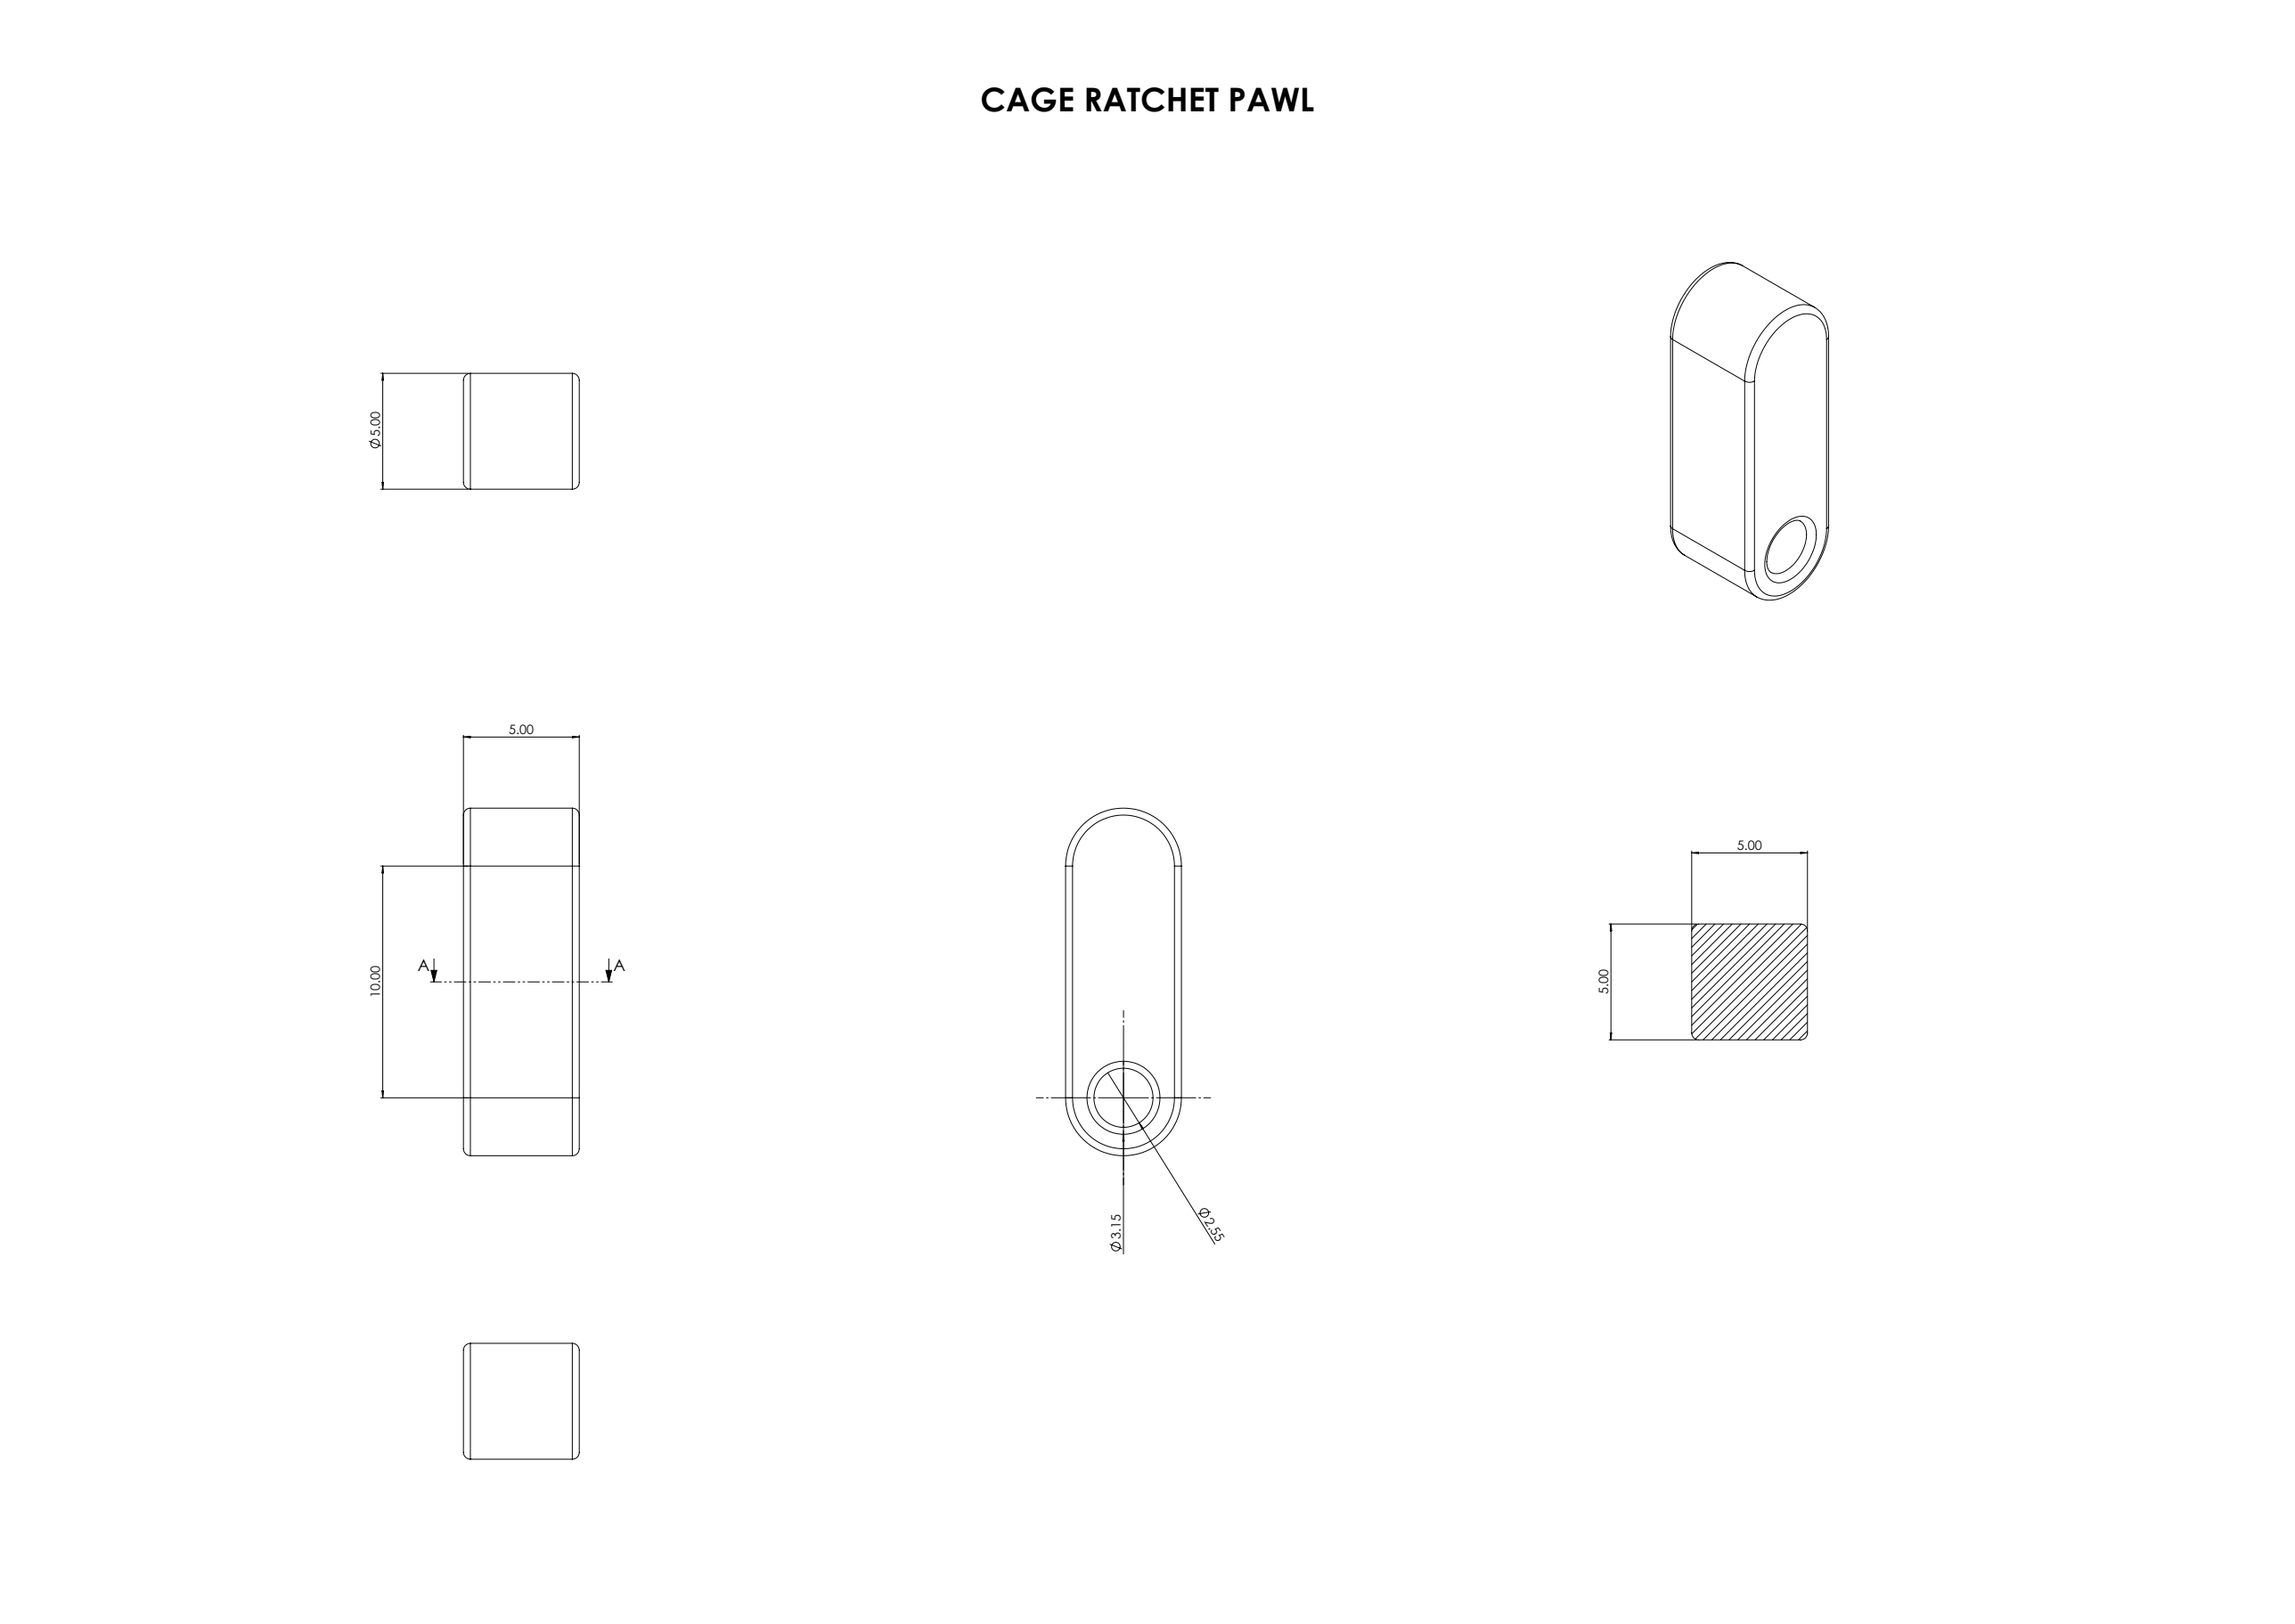
ISO-10303-21;
HEADER;
/* Generated by software containing ST-Developer
 * from STEP Tools, Inc. (www.steptools.com) 
 */

FILE_DESCRIPTION(
/* description */ (''),
/* implementation_level */ '2;1');

FILE_NAME(
/* name */ '05_Cage_Ratchet_Pawl.step',
/* time_stamp */ '2026-10-11T13:00:10-07:00',
/* author */ (''),
/* organization */ (''),
/* preprocessor_version */ 'ST-DEVELOPER v20.2',
/* originating_system */ 'Autodesk Translation Framework v15.15.0.0',
/* authorisation */ '');

FILE_SCHEMA (('AUTOMOTIVE_DESIGN { 1 0 10303 214 3 1 1 }'));
ENDSEC;

DATA;
#10=MECHANICAL_DESIGN_GEOMETRIC_PRESENTATION_REPRESENTATION('',(#362),#65563);
#149=TOROIDAL_SURFACE('',#21705,2.2,0.3);
#150=TOROIDAL_SURFACE('',#21711,2.2,0.3);
#151=TOROIDAL_SURFACE('',#21722,2.2,0.3);
#152=TOROIDAL_SURFACE('',#21728,2.2,0.3);
#153=TOROIDAL_SURFACE('',#21733,1.575,0.3);
#154=TOROIDAL_SURFACE('',#21739,1.575,0.3);
#340=SHAPE_REPRESENTATION_RELATIONSHIP('SRR','None',#65618,#351);
#351=ADVANCED_BREP_SHAPE_REPRESENTATION('',(#373),#65556);
#362=STYLED_ITEM('',(#65781),#373);
#373=MANIFOLD_SOLID_BREP('Body1',#20012);
#976=PLANE('',#21716);
#977=PLANE('',#21717);
#978=PLANE('',#21731);
#979=PLANE('',#21741);
#1118=FACE_BOUND('',#3216,.T.);
#1119=FACE_BOUND('',#3223,.T.);
#1987=FACE_OUTER_BOUND('',#3209,.T.);
#1988=FACE_OUTER_BOUND('',#3210,.T.);
#1989=FACE_OUTER_BOUND('',#3211,.T.);
#1990=FACE_OUTER_BOUND('',#3212,.T.);
#1991=FACE_OUTER_BOUND('',#3213,.T.);
#1992=FACE_OUTER_BOUND('',#3214,.T.);
#1993=FACE_OUTER_BOUND('',#3215,.T.);
#1994=FACE_OUTER_BOUND('',#3217,.T.);
#1995=FACE_OUTER_BOUND('',#3218,.T.);
#1996=FACE_OUTER_BOUND('',#3219,.T.);
#1997=FACE_OUTER_BOUND('',#3220,.T.);
#1998=FACE_OUTER_BOUND('',#3221,.T.);
#1999=FACE_OUTER_BOUND('',#3222,.T.);
#2000=FACE_OUTER_BOUND('',#3224,.T.);
#2001=FACE_OUTER_BOUND('',#3225,.T.);
#2002=FACE_OUTER_BOUND('',#3226,.T.);
#2003=FACE_OUTER_BOUND('',#3227,.T.);
#3209=EDGE_LOOP('',(#16744,#16745,#16746,#16747));
#3210=EDGE_LOOP('',(#16748,#16749,#16750,#16751));
#3211=EDGE_LOOP('',(#16752,#16753,#16754,#16755));
#3212=EDGE_LOOP('',(#16756,#16757,#16758,#16759));
#3213=EDGE_LOOP('',(#16760,#16761,#16762,#16763));
#3214=EDGE_LOOP('',(#16764,#16765,#16766,#16767));
#3215=EDGE_LOOP('',(#16768,#16769,#16770,#16771));
#3216=EDGE_LOOP('',(#16772));
#3217=EDGE_LOOP('',(#16773,#16774,#16775,#16776));
#3218=EDGE_LOOP('',(#16777,#16778,#16779,#16780));
#3219=EDGE_LOOP('',(#16781,#16782,#16783,#16784));
#3220=EDGE_LOOP('',(#16785,#16786,#16787,#16788));
#3221=EDGE_LOOP('',(#16789,#16790,#16791,#16792));
#3222=EDGE_LOOP('',(#16793,#16794,#16795,#16796));
#3223=EDGE_LOOP('',(#16797));
#3224=EDGE_LOOP('',(#16798,#16799,#16800,#16801));
#3225=EDGE_LOOP('',(#16802,#16803,#16804,#16805,#16806));
#3226=EDGE_LOOP('',(#16807,#16808,#16809,#16810,#16811));
#3227=EDGE_LOOP('',(#16812,#16813,#16814,#16815));
#4320=CIRCLE('',#21703,0.3);
#4321=CIRCLE('',#21704,0.3);
#4322=CIRCLE('',#21706,0.3);
#4323=CIRCLE('',#21707,2.2);
#4324=CIRCLE('',#21708,2.5);
#4325=CIRCLE('',#21710,0.3);
#4326=CIRCLE('',#21712,2.2);
#4327=CIRCLE('',#21713,2.5);
#4328=CIRCLE('',#21715,2.5);
#4329=CIRCLE('',#21718,1.575);
#4330=CIRCLE('',#21720,0.3);
#4331=CIRCLE('',#21721,0.3);
#4332=CIRCLE('',#21723,0.3);
#4333=CIRCLE('',#21724,2.2);
#4334=CIRCLE('',#21725,2.5);
#4335=CIRCLE('',#21727,0.3);
#4336=CIRCLE('',#21729,2.2);
#4337=CIRCLE('',#21732,1.575);
#4338=CIRCLE('',#21734,0.3);
#4339=CIRCLE('',#21735,1.275);
#4340=CIRCLE('',#21737,1.275);
#4341=CIRCLE('',#21738,1.275);
#4342=CIRCLE('',#21740,0.3);
#6010=LINE('',#61877,#6902);
#6011=LINE('',#61880,#6903);
#6012=LINE('',#61891,#6904);
#6013=LINE('',#61892,#6905);
#6014=LINE('',#61898,#6906);
#6015=LINE('',#61901,#6907);
#6016=LINE('',#61904,#6908);
#6017=LINE('',#61905,#6909);
#6018=LINE('',#61914,#6910);
#6019=LINE('',#61924,#6911);
#6020=LINE('',#61925,#6912);
#6021=LINE('',#61929,#6913);
#6022=LINE('',#61939,#6914);
#6902=VECTOR('',#26097,10.);
#6903=VECTOR('',#26100,10.);
#6904=VECTOR('',#26113,10.);
#6905=VECTOR('',#26114,10.);
#6906=VECTOR('',#26123,10.);
#6907=VECTOR('',#26126,10.);
#6908=VECTOR('',#26129,10.);
#6909=VECTOR('',#26130,10.);
#6910=VECTOR('',#26141,10.);
#6911=VECTOR('',#26154,10.);
#6912=VECTOR('',#26155,10.);
#6913=VECTOR('',#26162,10.);
#6914=VECTOR('',#26175,1.275);
#8661=VERTEX_POINT('',#61873);
#8662=VERTEX_POINT('',#61874);
#8663=VERTEX_POINT('',#61876);
#8664=VERTEX_POINT('',#61878);
#8665=VERTEX_POINT('',#61882);
#8666=VERTEX_POINT('',#61883);
#8667=VERTEX_POINT('',#61888);
#8668=VERTEX_POINT('',#61889);
#8669=VERTEX_POINT('',#61897);
#8670=VERTEX_POINT('',#61899);
#8671=VERTEX_POINT('',#61903);
#8672=VERTEX_POINT('',#61907);
#8673=VERTEX_POINT('',#61910);
#8674=VERTEX_POINT('',#61912);
#8675=VERTEX_POINT('',#61916);
#8676=VERTEX_POINT('',#61917);
#8677=VERTEX_POINT('',#61922);
#8678=VERTEX_POINT('',#61931);
#8679=VERTEX_POINT('',#61934);
#8680=VERTEX_POINT('',#61938);
#8681=VERTEX_POINT('',#61940);
#11405=EDGE_CURVE('',#8661,#8662,#4320,.T.);
#11406=EDGE_CURVE('',#8662,#8663,#6010,.T.);
#11407=EDGE_CURVE('',#8663,#8664,#4321,.T.);
#11408=EDGE_CURVE('',#8664,#8661,#6011,.T.);
#11409=EDGE_CURVE('',#8665,#8666,#4322,.T.);
#11410=EDGE_CURVE('',#8666,#8664,#4323,.T.);
#11411=EDGE_CURVE('',#8663,#8665,#4324,.T.);
#11412=EDGE_CURVE('',#8667,#8668,#4325,.T.);
#11413=EDGE_CURVE('',#8668,#8666,#6012,.T.);
#11414=EDGE_CURVE('',#8665,#8667,#6013,.T.);
#11415=EDGE_CURVE('',#8661,#8668,#4326,.T.);
#11416=EDGE_CURVE('',#8667,#8662,#4327,.T.);
#11417=EDGE_CURVE('',#8669,#8663,#6014,.T.);
#11418=EDGE_CURVE('',#8670,#8669,#4328,.T.);
#11419=EDGE_CURVE('',#8670,#8665,#6015,.T.);
#11420=EDGE_CURVE('',#8671,#8662,#6016,.T.);
#11421=EDGE_CURVE('',#8669,#8671,#6017,.T.);
#11422=EDGE_CURVE('',#8672,#8672,#4329,.T.);
#11423=EDGE_CURVE('',#8673,#8669,#4330,.T.);
#11424=EDGE_CURVE('',#8671,#8674,#4331,.T.);
#11425=EDGE_CURVE('',#8674,#8673,#6018,.T.);
#11426=EDGE_CURVE('',#8675,#8676,#4332,.T.);
#11427=EDGE_CURVE('',#8676,#8674,#4333,.T.);
#11428=EDGE_CURVE('',#8671,#8675,#4334,.T.);
#11429=EDGE_CURVE('',#8670,#8677,#4335,.T.);
#11430=EDGE_CURVE('',#8677,#8676,#6019,.T.);
#11431=EDGE_CURVE('',#8675,#8670,#6020,.T.);
#11432=EDGE_CURVE('',#8673,#8677,#4336,.T.);
#11433=EDGE_CURVE('',#8675,#8667,#6021,.T.);
#11434=EDGE_CURVE('',#8678,#8678,#4337,.T.);
#11435=EDGE_CURVE('',#8678,#8679,#4338,.T.);
#11436=EDGE_CURVE('',#8679,#8679,#4339,.T.);
#11437=EDGE_CURVE('',#8679,#8680,#6022,.T.);
#11438=EDGE_CURVE('',#8681,#8680,#4340,.T.);
#11439=EDGE_CURVE('',#8680,#8681,#4341,.T.);
#11440=EDGE_CURVE('',#8672,#8681,#4342,.T.);
#16744=ORIENTED_EDGE('',*,*,#11405,.T.);
#16745=ORIENTED_EDGE('',*,*,#11406,.T.);
#16746=ORIENTED_EDGE('',*,*,#11407,.T.);
#16747=ORIENTED_EDGE('',*,*,#11408,.T.);
#16748=ORIENTED_EDGE('',*,*,#11409,.T.);
#16749=ORIENTED_EDGE('',*,*,#11410,.T.);
#16750=ORIENTED_EDGE('',*,*,#11407,.F.);
#16751=ORIENTED_EDGE('',*,*,#11411,.T.);
#16752=ORIENTED_EDGE('',*,*,#11412,.T.);
#16753=ORIENTED_EDGE('',*,*,#11413,.T.);
#16754=ORIENTED_EDGE('',*,*,#11409,.F.);
#16755=ORIENTED_EDGE('',*,*,#11414,.T.);
#16756=ORIENTED_EDGE('',*,*,#11405,.F.);
#16757=ORIENTED_EDGE('',*,*,#11415,.T.);
#16758=ORIENTED_EDGE('',*,*,#11412,.F.);
#16759=ORIENTED_EDGE('',*,*,#11416,.T.);
#16760=ORIENTED_EDGE('',*,*,#11411,.F.);
#16761=ORIENTED_EDGE('',*,*,#11417,.F.);
#16762=ORIENTED_EDGE('',*,*,#11418,.F.);
#16763=ORIENTED_EDGE('',*,*,#11419,.T.);
#16764=ORIENTED_EDGE('',*,*,#11406,.F.);
#16765=ORIENTED_EDGE('',*,*,#11420,.F.);
#16766=ORIENTED_EDGE('',*,*,#11421,.F.);
#16767=ORIENTED_EDGE('',*,*,#11417,.T.);
#16768=ORIENTED_EDGE('',*,*,#11408,.F.);
#16769=ORIENTED_EDGE('',*,*,#11410,.F.);
#16770=ORIENTED_EDGE('',*,*,#11413,.F.);
#16771=ORIENTED_EDGE('',*,*,#11415,.F.);
#16772=ORIENTED_EDGE('',*,*,#11422,.F.);
#16773=ORIENTED_EDGE('',*,*,#11423,.T.);
#16774=ORIENTED_EDGE('',*,*,#11421,.T.);
#16775=ORIENTED_EDGE('',*,*,#11424,.T.);
#16776=ORIENTED_EDGE('',*,*,#11425,.T.);
#16777=ORIENTED_EDGE('',*,*,#11426,.T.);
#16778=ORIENTED_EDGE('',*,*,#11427,.T.);
#16779=ORIENTED_EDGE('',*,*,#11424,.F.);
#16780=ORIENTED_EDGE('',*,*,#11428,.T.);
#16781=ORIENTED_EDGE('',*,*,#11429,.T.);
#16782=ORIENTED_EDGE('',*,*,#11430,.T.);
#16783=ORIENTED_EDGE('',*,*,#11426,.F.);
#16784=ORIENTED_EDGE('',*,*,#11431,.T.);
#16785=ORIENTED_EDGE('',*,*,#11429,.F.);
#16786=ORIENTED_EDGE('',*,*,#11418,.T.);
#16787=ORIENTED_EDGE('',*,*,#11423,.F.);
#16788=ORIENTED_EDGE('',*,*,#11432,.T.);
#16789=ORIENTED_EDGE('',*,*,#11416,.F.);
#16790=ORIENTED_EDGE('',*,*,#11433,.F.);
#16791=ORIENTED_EDGE('',*,*,#11428,.F.);
#16792=ORIENTED_EDGE('',*,*,#11420,.T.);
#16793=ORIENTED_EDGE('',*,*,#11425,.F.);
#16794=ORIENTED_EDGE('',*,*,#11427,.F.);
#16795=ORIENTED_EDGE('',*,*,#11430,.F.);
#16796=ORIENTED_EDGE('',*,*,#11432,.F.);
#16797=ORIENTED_EDGE('',*,*,#11434,.F.);
#16798=ORIENTED_EDGE('',*,*,#11434,.T.);
#16799=ORIENTED_EDGE('',*,*,#11435,.T.);
#16800=ORIENTED_EDGE('',*,*,#11436,.T.);
#16801=ORIENTED_EDGE('',*,*,#11435,.F.);
#16802=ORIENTED_EDGE('',*,*,#11436,.F.);
#16803=ORIENTED_EDGE('',*,*,#11437,.T.);
#16804=ORIENTED_EDGE('',*,*,#11438,.F.);
#16805=ORIENTED_EDGE('',*,*,#11439,.F.);
#16806=ORIENTED_EDGE('',*,*,#11437,.F.);
#16807=ORIENTED_EDGE('',*,*,#11422,.T.);
#16808=ORIENTED_EDGE('',*,*,#11440,.T.);
#16809=ORIENTED_EDGE('',*,*,#11438,.T.);
#16810=ORIENTED_EDGE('',*,*,#11439,.T.);
#16811=ORIENTED_EDGE('',*,*,#11440,.F.);
#16812=ORIENTED_EDGE('',*,*,#11414,.F.);
#16813=ORIENTED_EDGE('',*,*,#11419,.F.);
#16814=ORIENTED_EDGE('',*,*,#11431,.F.);
#16815=ORIENTED_EDGE('',*,*,#11433,.T.);
#18717=CYLINDRICAL_SURFACE('',#21702,0.3);
#18718=CYLINDRICAL_SURFACE('',#21709,0.3);
#18719=CYLINDRICAL_SURFACE('',#21714,2.5);
#18720=CYLINDRICAL_SURFACE('',#21719,0.3);
#18721=CYLINDRICAL_SURFACE('',#21726,0.3);
#18722=CYLINDRICAL_SURFACE('',#21730,2.5);
#18723=CYLINDRICAL_SURFACE('',#21736,1.275);
#19683=ADVANCED_FACE('',(#1987),#18717,.T.);
#19684=ADVANCED_FACE('',(#1988),#149,.T.);
#19685=ADVANCED_FACE('',(#1989),#18718,.T.);
#19686=ADVANCED_FACE('',(#1990),#150,.T.);
#19687=ADVANCED_FACE('',(#1991),#18719,.T.);
#19688=ADVANCED_FACE('',(#1992),#976,.T.);
#19689=ADVANCED_FACE('',(#1993,#1118),#977,.T.);
#19690=ADVANCED_FACE('',(#1994),#18720,.T.);
#19691=ADVANCED_FACE('',(#1995),#151,.T.);
#19692=ADVANCED_FACE('',(#1996),#18721,.T.);
#19693=ADVANCED_FACE('',(#1997),#152,.T.);
#19694=ADVANCED_FACE('',(#1998),#18722,.T.);
#19695=ADVANCED_FACE('',(#1999,#1119),#978,.F.);
#19696=ADVANCED_FACE('',(#2000),#153,.T.);
#19697=ADVANCED_FACE('',(#2001),#18723,.F.);
#19698=ADVANCED_FACE('',(#2002),#154,.T.);
#19699=ADVANCED_FACE('',(#2003),#979,.T.);
#20012=CLOSED_SHELL('',(#19683,#19684,#19685,#19686,#19687,#19688,#19689,
#19690,#19691,#19692,#19693,#19694,#19695,#19696,#19697,#19698,#19699));
#21701=AXIS2_PLACEMENT_3D('',#61871,#26091,#26092);
#21702=AXIS2_PLACEMENT_3D('',#61872,#26093,#26094);
#21703=AXIS2_PLACEMENT_3D('',#61875,#26095,#26096);
#21704=AXIS2_PLACEMENT_3D('',#61879,#26098,#26099);
#21705=AXIS2_PLACEMENT_3D('',#61881,#26101,#26102);
#21706=AXIS2_PLACEMENT_3D('',#61884,#26103,#26104);
#21707=AXIS2_PLACEMENT_3D('',#61885,#26105,#26106);
#21708=AXIS2_PLACEMENT_3D('',#61886,#26107,#26108);
#21709=AXIS2_PLACEMENT_3D('',#61887,#26109,#26110);
#21710=AXIS2_PLACEMENT_3D('',#61890,#26111,#26112);
#21711=AXIS2_PLACEMENT_3D('',#61893,#26115,#26116);
#21712=AXIS2_PLACEMENT_3D('',#61894,#26117,#26118);
#21713=AXIS2_PLACEMENT_3D('',#61895,#26119,#26120);
#21714=AXIS2_PLACEMENT_3D('',#61896,#26121,#26122);
#21715=AXIS2_PLACEMENT_3D('',#61900,#26124,#26125);
#21716=AXIS2_PLACEMENT_3D('',#61902,#26127,#26128);
#21717=AXIS2_PLACEMENT_3D('',#61906,#26131,#26132);
#21718=AXIS2_PLACEMENT_3D('',#61908,#26133,#26134);
#21719=AXIS2_PLACEMENT_3D('',#61909,#26135,#26136);
#21720=AXIS2_PLACEMENT_3D('',#61911,#26137,#26138);
#21721=AXIS2_PLACEMENT_3D('',#61913,#26139,#26140);
#21722=AXIS2_PLACEMENT_3D('',#61915,#26142,#26143);
#21723=AXIS2_PLACEMENT_3D('',#61918,#26144,#26145);
#21724=AXIS2_PLACEMENT_3D('',#61919,#26146,#26147);
#21725=AXIS2_PLACEMENT_3D('',#61920,#26148,#26149);
#21726=AXIS2_PLACEMENT_3D('',#61921,#26150,#26151);
#21727=AXIS2_PLACEMENT_3D('',#61923,#26152,#26153);
#21728=AXIS2_PLACEMENT_3D('',#61926,#26156,#26157);
#21729=AXIS2_PLACEMENT_3D('',#61927,#26158,#26159);
#21730=AXIS2_PLACEMENT_3D('',#61928,#26160,#26161);
#21731=AXIS2_PLACEMENT_3D('',#61930,#26163,#26164);
#21732=AXIS2_PLACEMENT_3D('',#61932,#26165,#26166);
#21733=AXIS2_PLACEMENT_3D('',#61933,#26167,#26168);
#21734=AXIS2_PLACEMENT_3D('',#61935,#26169,#26170);
#21735=AXIS2_PLACEMENT_3D('',#61936,#26171,#26172);
#21736=AXIS2_PLACEMENT_3D('',#61937,#26173,#26174);
#21737=AXIS2_PLACEMENT_3D('',#61941,#26176,#26177);
#21738=AXIS2_PLACEMENT_3D('',#61942,#26178,#26179);
#21739=AXIS2_PLACEMENT_3D('',#61943,#26180,#26181);
#21740=AXIS2_PLACEMENT_3D('',#61944,#26182,#26183);
#21741=AXIS2_PLACEMENT_3D('',#61945,#26184,#26185);
#26091=DIRECTION('axis',(0.,0.,1.));
#26092=DIRECTION('refdir',(1.,0.,0.));
#26093=DIRECTION('center_axis',(0.,-1.,0.));
#26094=DIRECTION('ref_axis',(0.707106781186548,0.,0.707106781186547));
#26095=DIRECTION('center_axis',(0.,-1.,0.));
#26096=DIRECTION('ref_axis',(1.,0.,0.));
#26097=DIRECTION('',(0.,-1.,0.));
#26098=DIRECTION('center_axis',(0.,1.,0.));
#26099=DIRECTION('ref_axis',(0.,0.,1.));
#26100=DIRECTION('',(0.,1.,0.));
#26101=DIRECTION('center_axis',(1.,0.,0.));
#26102=DIRECTION('ref_axis',(0.,0.,-1.));
#26103=DIRECTION('center_axis',(0.,-1.,0.));
#26104=DIRECTION('ref_axis',(0.,0.,-1.));
#26105=DIRECTION('center_axis',(-1.,0.,0.));
#26106=DIRECTION('ref_axis',(0.,-1.,-6.12323399573677E-17));
#26107=DIRECTION('center_axis',(1.,0.,0.));
#26108=DIRECTION('ref_axis',(0.,-1.,-6.12323399573677E-17));
#26109=DIRECTION('center_axis',(0.,1.,0.));
#26110=DIRECTION('ref_axis',(0.707106781186548,0.,-0.707106781186547));
#26111=DIRECTION('center_axis',(0.,-1.,0.));
#26112=DIRECTION('ref_axis',(0.,0.,-1.));
#26113=DIRECTION('',(0.,-1.,0.));
#26114=DIRECTION('',(0.,1.,0.));
#26115=DIRECTION('center_axis',(1.,0.,0.));
#26116=DIRECTION('ref_axis',(0.,0.,-1.));
#26117=DIRECTION('center_axis',(-1.,0.,0.));
#26118=DIRECTION('ref_axis',(0.,1.,-6.12323399573677E-17));
#26119=DIRECTION('center_axis',(1.,0.,0.));
#26120=DIRECTION('ref_axis',(0.,1.,-6.12323399573677E-17));
#26121=DIRECTION('center_axis',(1.,0.,0.));
#26122=DIRECTION('ref_axis',(0.,0.,-1.));
#26123=DIRECTION('',(1.,0.,0.));
#26124=DIRECTION('center_axis',(-1.,0.,0.));
#26125=DIRECTION('ref_axis',(0.,-1.,-6.12323399573677E-17));
#26126=DIRECTION('',(1.,0.,0.));
#26127=DIRECTION('center_axis',(0.,0.,1.));
#26128=DIRECTION('ref_axis',(0.,-1.,0.));
#26129=DIRECTION('',(1.,0.,0.));
#26130=DIRECTION('',(0.,1.,0.));
#26131=DIRECTION('center_axis',(1.,0.,0.));
#26132=DIRECTION('ref_axis',(0.,0.,-1.));
#26133=DIRECTION('center_axis',(1.,0.,0.));
#26134=DIRECTION('ref_axis',(0.,0.,-1.));
#26135=DIRECTION('center_axis',(0.,1.,0.));
#26136=DIRECTION('ref_axis',(-0.707106781186548,0.,0.707106781186547));
#26137=DIRECTION('center_axis',(0.,1.,0.));
#26138=DIRECTION('ref_axis',(-1.,0.,0.));
#26139=DIRECTION('center_axis',(0.,-1.,0.));
#26140=DIRECTION('ref_axis',(0.,0.,1.));
#26141=DIRECTION('',(0.,-1.,0.));
#26142=DIRECTION('center_axis',(1.,0.,0.));
#26143=DIRECTION('ref_axis',(0.,0.,-1.));
#26144=DIRECTION('center_axis',(0.,1.,0.));
#26145=DIRECTION('ref_axis',(0.,0.,-1.));
#26146=DIRECTION('center_axis',(1.,0.,0.));
#26147=DIRECTION('ref_axis',(0.,1.,-6.12323399573677E-17));
#26148=DIRECTION('center_axis',(-1.,0.,0.));
#26149=DIRECTION('ref_axis',(0.,1.,-6.12323399573677E-17));
#26150=DIRECTION('center_axis',(0.,-1.,0.));
#26151=DIRECTION('ref_axis',(-0.707106781186548,0.,-0.707106781186547));
#26152=DIRECTION('center_axis',(0.,1.,0.));
#26153=DIRECTION('ref_axis',(0.,0.,-1.));
#26154=DIRECTION('',(0.,1.,0.));
#26155=DIRECTION('',(0.,-1.,0.));
#26156=DIRECTION('center_axis',(1.,0.,0.));
#26157=DIRECTION('ref_axis',(0.,0.,-1.));
#26158=DIRECTION('center_axis',(1.,0.,0.));
#26159=DIRECTION('ref_axis',(0.,-1.,-6.12323399573677E-17));
#26160=DIRECTION('center_axis',(1.,0.,0.));
#26161=DIRECTION('ref_axis',(0.,0.,-1.));
#26162=DIRECTION('',(1.,0.,0.));
#26163=DIRECTION('center_axis',(1.,0.,0.));
#26164=DIRECTION('ref_axis',(0.,0.,-1.));
#26165=DIRECTION('center_axis',(-1.,0.,0.));
#26166=DIRECTION('ref_axis',(0.,0.,-1.));
#26167=DIRECTION('center_axis',(1.,0.,0.));
#26168=DIRECTION('ref_axis',(0.,0.,-1.));
#26169=DIRECTION('center_axis',(0.,-1.,-1.22464679914735E-16));
#26170=DIRECTION('ref_axis',(0.,-1.22464679914735E-16,1.));
#26171=DIRECTION('center_axis',(1.,0.,0.));
#26172=DIRECTION('ref_axis',(0.,0.,-1.));
#26173=DIRECTION('center_axis',(1.,0.,0.));
#26174=DIRECTION('ref_axis',(0.,0.,-1.));
#26175=DIRECTION('',(1.,0.,0.));
#26176=DIRECTION('center_axis',(-1.,0.,0.));
#26177=DIRECTION('ref_axis',(0.,0.,-1.));
#26178=DIRECTION('center_axis',(-1.,0.,0.));
#26179=DIRECTION('ref_axis',(0.,0.,-1.));
#26180=DIRECTION('center_axis',(-1.,0.,0.));
#26181=DIRECTION('ref_axis',(0.,0.,1.));
#26182=DIRECTION('center_axis',(0.,-1.,1.22464679914735E-16));
#26183=DIRECTION('ref_axis',(0.,-1.22464679914735E-16,-1.));
#26184=DIRECTION('center_axis',(0.,0.,-1.));
#26185=DIRECTION('ref_axis',(0.,1.,0.));
#61871=CARTESIAN_POINT('',(0.,0.,0.));
#61872=CARTESIAN_POINT('Origin',(4.7,7.5,2.2));
#61873=CARTESIAN_POINT('',(5.,10.,2.2));
#61874=CARTESIAN_POINT('',(4.7,10.,2.5));
#61875=CARTESIAN_POINT('Origin',(4.7,10.,2.2));
#61876=CARTESIAN_POINT('',(4.7,0.,2.5));
#61877=CARTESIAN_POINT('',(4.7,7.5,2.5));
#61878=CARTESIAN_POINT('',(5.,0.,2.2));
#61879=CARTESIAN_POINT('Origin',(4.7,0.,2.2));
#61880=CARTESIAN_POINT('',(5.,7.5,2.2));
#61881=CARTESIAN_POINT('Origin',(4.7,0.,0.));
#61882=CARTESIAN_POINT('',(4.7,0.,-2.5));
#61883=CARTESIAN_POINT('',(5.,0.,-2.2));
#61884=CARTESIAN_POINT('Origin',(4.7,0.,-2.2));
#61885=CARTESIAN_POINT('Origin',(5.,0.,0.));
#61886=CARTESIAN_POINT('Origin',(4.7,0.,0.));
#61887=CARTESIAN_POINT('Origin',(4.7,2.5,-2.2));
#61888=CARTESIAN_POINT('',(4.7,10.,-2.5));
#61889=CARTESIAN_POINT('',(5.,10.,-2.2));
#61890=CARTESIAN_POINT('Origin',(4.7,10.,-2.2));
#61891=CARTESIAN_POINT('',(5.,2.5,-2.2));
#61892=CARTESIAN_POINT('',(4.7,2.5,-2.5));
#61893=CARTESIAN_POINT('Origin',(4.7,10.,0.));
#61894=CARTESIAN_POINT('Origin',(5.,10.,0.));
#61895=CARTESIAN_POINT('Origin',(4.7,10.,0.));
#61896=CARTESIAN_POINT('Origin',(0.,0.,0.));
#61897=CARTESIAN_POINT('',(0.3,0.,2.5));
#61898=CARTESIAN_POINT('',(0.,0.,2.5));
#61899=CARTESIAN_POINT('',(0.3,0.,-2.5));
#61900=CARTESIAN_POINT('Origin',(0.3,0.,0.));
#61901=CARTESIAN_POINT('',(0.,0.,-2.5));
#61902=CARTESIAN_POINT('Origin',(0.,10.,2.5));
#61903=CARTESIAN_POINT('',(0.3,10.,2.5));
#61904=CARTESIAN_POINT('',(0.,10.,2.5));
#61905=CARTESIAN_POINT('',(0.3,7.5,2.5));
#61906=CARTESIAN_POINT('Origin',(5.,5.,0.));
#61907=CARTESIAN_POINT('',(5.,-1.92881870865708E-16,-1.575));
#61908=CARTESIAN_POINT('Origin',(5.,0.,0.));
#61909=CARTESIAN_POINT('Origin',(0.3,7.5,2.2));
#61910=CARTESIAN_POINT('',(0.,0.,2.2));
#61911=CARTESIAN_POINT('Origin',(0.3,0.,2.2));
#61912=CARTESIAN_POINT('',(0.,10.,2.2));
#61913=CARTESIAN_POINT('Origin',(0.3,10.,2.2));
#61914=CARTESIAN_POINT('',(0.,7.5,2.2));
#61915=CARTESIAN_POINT('Origin',(0.3,10.,0.));
#61916=CARTESIAN_POINT('',(0.3,10.,-2.5));
#61917=CARTESIAN_POINT('',(0.,10.,-2.2));
#61918=CARTESIAN_POINT('Origin',(0.3,10.,-2.2));
#61919=CARTESIAN_POINT('Origin',(0.,10.,0.));
#61920=CARTESIAN_POINT('Origin',(0.3,10.,0.));
#61921=CARTESIAN_POINT('Origin',(0.3,2.5,-2.2));
#61922=CARTESIAN_POINT('',(0.,0.,-2.2));
#61923=CARTESIAN_POINT('Origin',(0.3,0.,-2.2));
#61924=CARTESIAN_POINT('',(0.,2.5,-2.2));
#61925=CARTESIAN_POINT('',(0.3,2.5,-2.5));
#61926=CARTESIAN_POINT('Origin',(0.3,0.,0.));
#61927=CARTESIAN_POINT('Origin',(0.,0.,0.));
#61928=CARTESIAN_POINT('Origin',(0.,10.,0.));
#61929=CARTESIAN_POINT('',(0.,10.,-2.5));
#61930=CARTESIAN_POINT('Origin',(0.,5.,0.));
#61931=CARTESIAN_POINT('',(0.,1.92881870865708E-16,1.575));
#61932=CARTESIAN_POINT('Origin',(0.,0.,0.));
#61933=CARTESIAN_POINT('Origin',(0.3,0.,0.));
#61934=CARTESIAN_POINT('',(0.3,-1.56142466891288E-16,1.275));
#61935=CARTESIAN_POINT('Origin',(0.3,-1.92881870865708E-16,1.575));
#61936=CARTESIAN_POINT('Origin',(0.3,0.,0.));
#61937=CARTESIAN_POINT('Origin',(0.,0.,0.));
#61938=CARTESIAN_POINT('',(4.7,1.56142466891288E-16,1.275));
#61939=CARTESIAN_POINT('',(0.,-1.56142466891288E-16,1.275));
#61940=CARTESIAN_POINT('',(4.7,-1.56142466891288E-16,-1.275));
#61941=CARTESIAN_POINT('Origin',(4.7,0.,0.));
#61942=CARTESIAN_POINT('Origin',(4.7,0.,0.));
#61943=CARTESIAN_POINT('Origin',(4.7,0.,0.));
#61944=CARTESIAN_POINT('Origin',(4.7,-1.92881870865708E-16,-1.575));
#61945=CARTESIAN_POINT('Origin',(0.,0.,-2.5));
#65543=UNCERTAINTY_MEASURE_WITH_UNIT(LENGTH_MEASURE(0.01),#65564,
'DISTANCE_ACCURACY_VALUE',
'Maximum model space distance between geometric entities at asserted c
onnectivities');
#65550=UNCERTAINTY_MEASURE_WITH_UNIT(LENGTH_MEASURE(0.01),#65564,
'DISTANCE_ACCURACY_VALUE',
'Maximum model space distance between geometric entities at asserted c
onnectivities');
#65556=(
GEOMETRIC_REPRESENTATION_CONTEXT(3)
GLOBAL_UNCERTAINTY_ASSIGNED_CONTEXT((#65543))
GLOBAL_UNIT_ASSIGNED_CONTEXT((#65564,#65566,#65567))
REPRESENTATION_CONTEXT('','3D')
);
#65563=(
GEOMETRIC_REPRESENTATION_CONTEXT(3)
GLOBAL_UNCERTAINTY_ASSIGNED_CONTEXT((#65550))
GLOBAL_UNIT_ASSIGNED_CONTEXT((#65564,#65566,#65567))
REPRESENTATION_CONTEXT('','3D')
);
#65564=(
LENGTH_UNIT()
NAMED_UNIT(*)
SI_UNIT(.MILLI.,.METRE.)
);
#65566=(
NAMED_UNIT(*)
PLANE_ANGLE_UNIT()
SI_UNIT($,.RADIAN.)
);
#65567=(
NAMED_UNIT(*)
SI_UNIT($,.STERADIAN.)
SOLID_ANGLE_UNIT()
);
#65573=SHAPE_DEFINITION_REPRESENTATION(#65585,#65618);
#65585=PRODUCT_DEFINITION_SHAPE('',$,#65631);
#65618=SHAPE_REPRESENTATION('',(#21701),#65556);
#65625=PRODUCT_DEFINITION_CONTEXT('part definition',#65663,'design');
#65631=PRODUCT_DEFINITION('2026-10-10-05-45-27-787',
'05_Cage_Ratchet_Pawl',#65643,#65625);
#65643=PRODUCT_DEFINITION_FORMATION('',$,#65670);
#65663=APPLICATION_CONTEXT(
'Core Data for Automotive Mechanical Design Process');
#65664=PRODUCT_CONTEXT('part definition',#65663,'mechanical');
#65670=PRODUCT('2026-10-10-05-45-27-787','05_Cage_Ratchet_Pawl',$,(#65664));
#65775=COLOUR_RGB('Sky Blue',0.24,0.69,0.87);
#65776=FILL_AREA_STYLE_COLOUR('',#65775);
#65777=FILL_AREA_STYLE('',(#65776));
#65778=SURFACE_STYLE_FILL_AREA(#65777);
#65779=SURFACE_SIDE_STYLE('',(#65778));
#65780=SURFACE_STYLE_USAGE(.BOTH.,#65779);
#65781=PRESENTATION_STYLE_ASSIGNMENT((#65780));
ENDSEC;
END-ISO-10303-21;
